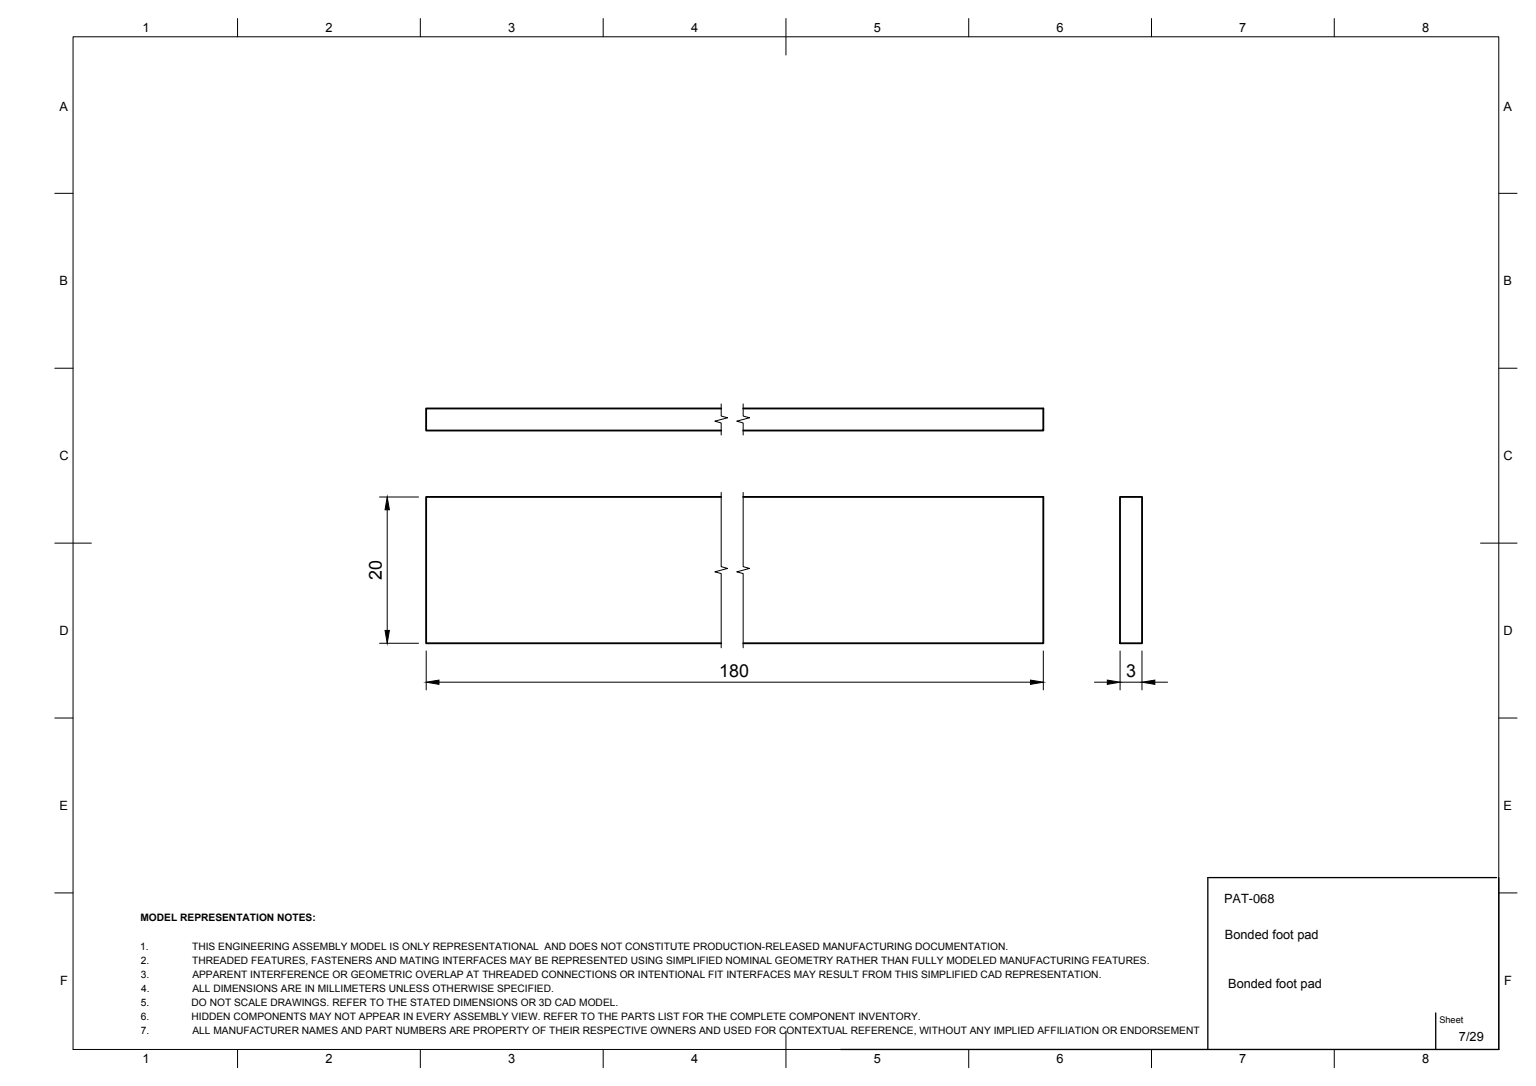
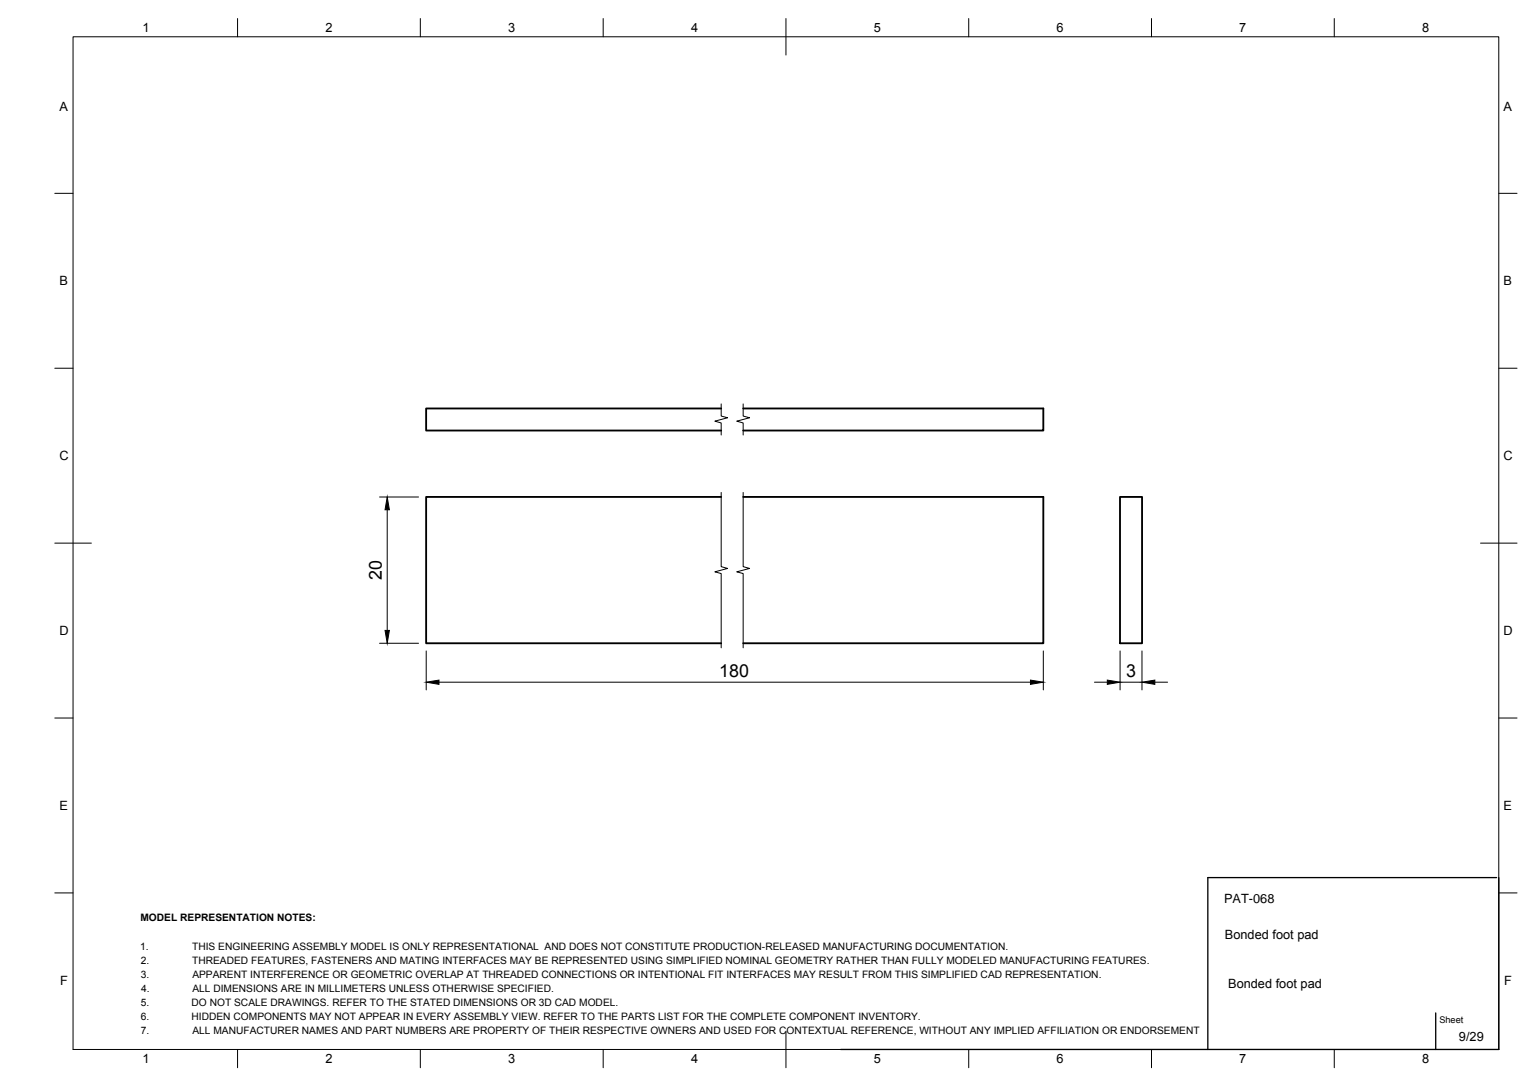
ISO-10303-21;
HEADER;
/* Generated by software containing ST-Developer
 * from STEP Tools, Inc. (www.steptools.com) 
 */

FILE_DESCRIPTION(
/* description */ ('Line shaft on three pillow blocks'),
/* implementation_level */ '2;1');

FILE_NAME(
/* name */ 'Bonded foot pad.step',
/* time_stamp */ '2026-10-27T10:49:19-07:00',
/* author */ (''),
/* organization */ (''),
/* preprocessor_version */ 'ST-DEVELOPER v20.2',
/* originating_system */ 'Autodesk Translation Framework v15.17.0.0',
/* authorisation */ '');

FILE_SCHEMA (('AUTOMOTIVE_DESIGN { 1 0 10303 214 3 1 1 }'));
ENDSEC;

DATA;
#10=MECHANICAL_DESIGN_GEOMETRIC_PRESENTATION_REPRESENTATION('',(#340),#8377);
#286=SHAPE_REPRESENTATION_RELATIONSHIP('SRR','None',#8501,#313);
#313=ADVANCED_BREP_SHAPE_REPRESENTATION('',(#368),#8350);
#340=STYLED_ITEM('',(#8711),#368);
#368=MANIFOLD_SOLID_BREP('Body1',#4326);
#502=PLANE('',#4708);
#503=PLANE('',#4709);
#504=PLANE('',#4710);
#505=PLANE('',#4711);
#506=PLANE('',#4712);
#507=PLANE('',#4713);
#680=FACE_OUTER_BOUND('',#954,.T.);
#681=FACE_OUTER_BOUND('',#955,.T.);
#682=FACE_OUTER_BOUND('',#956,.T.);
#683=FACE_OUTER_BOUND('',#957,.T.);
#684=FACE_OUTER_BOUND('',#958,.T.);
#685=FACE_OUTER_BOUND('',#959,.T.);
#954=EDGE_LOOP('',(#3069,#3070,#3071,#3072));
#955=EDGE_LOOP('',(#3073,#3074,#3075,#3076));
#956=EDGE_LOOP('',(#3077,#3078,#3079,#3080));
#957=EDGE_LOOP('',(#3081,#3082,#3083,#3084));
#958=EDGE_LOOP('',(#3085,#3086,#3087,#3088));
#959=EDGE_LOOP('',(#3089,#3090,#3091,#3092));
#1291=LINE('',#6599,#1618);
#1292=LINE('',#6601,#1619);
#1293=LINE('',#6603,#1620);
#1294=LINE('',#6604,#1621);
#1295=LINE('',#6607,#1622);
#1296=LINE('',#6609,#1623);
#1297=LINE('',#6610,#1624);
#1298=LINE('',#6613,#1625);
#1299=LINE('',#6615,#1626);
#1300=LINE('',#6616,#1627);
#1301=LINE('',#6618,#1628);
#1302=LINE('',#6619,#1629);
#1618=VECTOR('',#5296,1.);
#1619=VECTOR('',#5297,1.);
#1620=VECTOR('',#5298,1.);
#1621=VECTOR('',#5299,1.);
#1622=VECTOR('',#5302,1.);
#1623=VECTOR('',#5303,1.);
#1624=VECTOR('',#5304,1.);
#1625=VECTOR('',#5307,1.);
#1626=VECTOR('',#5308,1.);
#1627=VECTOR('',#5309,1.);
#1628=VECTOR('',#5312,1.);
#1629=VECTOR('',#5313,1.);
#2108=VERTEX_POINT('',#6597);
#2109=VERTEX_POINT('',#6598);
#2110=VERTEX_POINT('',#6600);
#2111=VERTEX_POINT('',#6602);
#2112=VERTEX_POINT('',#6606);
#2113=VERTEX_POINT('',#6608);
#2114=VERTEX_POINT('',#6612);
#2115=VERTEX_POINT('',#6614);
#2483=EDGE_CURVE('',#2108,#2109,#1291,.T.);
#2484=EDGE_CURVE('',#2109,#2110,#1292,.T.);
#2485=EDGE_CURVE('',#2111,#2110,#1293,.T.);
#2486=EDGE_CURVE('',#2108,#2111,#1294,.T.);
#2487=EDGE_CURVE('',#2112,#2108,#1295,.T.);
#2488=EDGE_CURVE('',#2113,#2111,#1296,.T.);
#2489=EDGE_CURVE('',#2112,#2113,#1297,.T.);
#2490=EDGE_CURVE('',#2114,#2112,#1298,.T.);
#2491=EDGE_CURVE('',#2115,#2113,#1299,.T.);
#2492=EDGE_CURVE('',#2114,#2115,#1300,.T.);
#2493=EDGE_CURVE('',#2109,#2114,#1301,.T.);
#2494=EDGE_CURVE('',#2110,#2115,#1302,.T.);
#3069=ORIENTED_EDGE('',*,*,#2483,.T.);
#3070=ORIENTED_EDGE('',*,*,#2484,.T.);
#3071=ORIENTED_EDGE('',*,*,#2485,.F.);
#3072=ORIENTED_EDGE('',*,*,#2486,.F.);
#3073=ORIENTED_EDGE('',*,*,#2487,.T.);
#3074=ORIENTED_EDGE('',*,*,#2486,.T.);
#3075=ORIENTED_EDGE('',*,*,#2488,.F.);
#3076=ORIENTED_EDGE('',*,*,#2489,.F.);
#3077=ORIENTED_EDGE('',*,*,#2490,.T.);
#3078=ORIENTED_EDGE('',*,*,#2489,.T.);
#3079=ORIENTED_EDGE('',*,*,#2491,.F.);
#3080=ORIENTED_EDGE('',*,*,#2492,.F.);
#3081=ORIENTED_EDGE('',*,*,#2493,.T.);
#3082=ORIENTED_EDGE('',*,*,#2492,.T.);
#3083=ORIENTED_EDGE('',*,*,#2494,.F.);
#3084=ORIENTED_EDGE('',*,*,#2484,.F.);
#3085=ORIENTED_EDGE('',*,*,#2494,.T.);
#3086=ORIENTED_EDGE('',*,*,#2491,.T.);
#3087=ORIENTED_EDGE('',*,*,#2488,.T.);
#3088=ORIENTED_EDGE('',*,*,#2485,.T.);
#3089=ORIENTED_EDGE('',*,*,#2493,.F.);
#3090=ORIENTED_EDGE('',*,*,#2483,.F.);
#3091=ORIENTED_EDGE('',*,*,#2487,.F.);
#3092=ORIENTED_EDGE('',*,*,#2490,.F.);
#4098=ADVANCED_FACE('',(#680),#502,.T.);
#4099=ADVANCED_FACE('',(#681),#503,.T.);
#4100=ADVANCED_FACE('',(#682),#504,.T.);
#4101=ADVANCED_FACE('',(#683),#505,.T.);
#4102=ADVANCED_FACE('',(#684),#506,.T.);
#4103=ADVANCED_FACE('',(#685),#507,.F.);
#4326=CLOSED_SHELL('',(#4098,#4099,#4100,#4101,#4102,#4103));
#4707=AXIS2_PLACEMENT_3D('',#6595,#5292,#5293);
#4708=AXIS2_PLACEMENT_3D('',#6596,#5294,#5295);
#4709=AXIS2_PLACEMENT_3D('',#6605,#5300,#5301);
#4710=AXIS2_PLACEMENT_3D('',#6611,#5305,#5306);
#4711=AXIS2_PLACEMENT_3D('',#6617,#5310,#5311);
#4712=AXIS2_PLACEMENT_3D('',#6620,#5314,#5315);
#4713=AXIS2_PLACEMENT_3D('',#6621,#5316,#5317);
#5292=DIRECTION('axis',(0.,0.,1.));
#5293=DIRECTION('refdir',(1.,0.,0.));
#5294=DIRECTION('center_axis',(0.,1.,0.));
#5295=DIRECTION('ref_axis',(-1.,0.,0.));
#5296=DIRECTION('',(-1.,0.,0.));
#5297=DIRECTION('',(0.,0.,1.));
#5298=DIRECTION('',(-1.,0.,0.));
#5299=DIRECTION('',(0.,0.,1.));
#5300=DIRECTION('center_axis',(1.,0.,0.));
#5301=DIRECTION('ref_axis',(0.,1.,0.));
#5302=DIRECTION('',(0.,1.,0.));
#5303=DIRECTION('',(0.,1.,0.));
#5304=DIRECTION('',(0.,0.,1.));
#5305=DIRECTION('center_axis',(0.,-1.,0.));
#5306=DIRECTION('ref_axis',(1.,0.,0.));
#5307=DIRECTION('',(1.,0.,0.));
#5308=DIRECTION('',(1.,0.,0.));
#5309=DIRECTION('',(0.,0.,1.));
#5310=DIRECTION('center_axis',(-1.,0.,0.));
#5311=DIRECTION('ref_axis',(0.,-1.,0.));
#5312=DIRECTION('',(0.,-1.,0.));
#5313=DIRECTION('',(0.,-1.,0.));
#5314=DIRECTION('center_axis',(0.,0.,1.));
#5315=DIRECTION('ref_axis',(1.,0.,0.));
#5316=DIRECTION('center_axis',(0.,0.,1.));
#5317=DIRECTION('ref_axis',(1.,0.,0.));
#6595=CARTESIAN_POINT('',(0.,0.,0.));
#6596=CARTESIAN_POINT('Origin',(9.,-2.,-1.8));
#6597=CARTESIAN_POINT('',(9.,-2.,-1.8));
#6598=CARTESIAN_POINT('',(-9.,-2.,-1.8));
#6599=CARTESIAN_POINT('',(9.,-2.,-1.8));
#6600=CARTESIAN_POINT('',(-9.,-2.,-1.5));
#6601=CARTESIAN_POINT('',(-9.,-2.,-1.8));
#6602=CARTESIAN_POINT('',(9.,-2.,-1.5));
#6603=CARTESIAN_POINT('',(9.,-2.,-1.5));
#6604=CARTESIAN_POINT('',(9.,-2.,-1.8));
#6605=CARTESIAN_POINT('Origin',(9.,-4.,-1.8));
#6606=CARTESIAN_POINT('',(9.,-4.,-1.8));
#6607=CARTESIAN_POINT('',(9.,-4.,-1.8));
#6608=CARTESIAN_POINT('',(9.,-4.,-1.5));
#6609=CARTESIAN_POINT('',(9.,-4.,-1.5));
#6610=CARTESIAN_POINT('',(9.,-4.,-1.8));
#6611=CARTESIAN_POINT('Origin',(-9.,-4.,-1.8));
#6612=CARTESIAN_POINT('',(-9.,-4.,-1.8));
#6613=CARTESIAN_POINT('',(-9.,-4.,-1.8));
#6614=CARTESIAN_POINT('',(-9.,-4.,-1.5));
#6615=CARTESIAN_POINT('',(-9.,-4.,-1.5));
#6616=CARTESIAN_POINT('',(-9.,-4.,-1.8));
#6617=CARTESIAN_POINT('Origin',(-9.,-2.,-1.8));
#6618=CARTESIAN_POINT('',(-9.,-2.,-1.8));
#6619=CARTESIAN_POINT('',(-9.,-2.,-1.5));
#6620=CARTESIAN_POINT('Origin',(0.,-3.,-1.5));
#6621=CARTESIAN_POINT('Origin',(0.,-3.,-1.8));
#8318=UNCERTAINTY_MEASURE_WITH_UNIT(LENGTH_MEASURE(0.001),#8378,
'DISTANCE_ACCURACY_VALUE',
'Maximum model space distance between geometric entities at asserted c
onnectivities');
#8345=UNCERTAINTY_MEASURE_WITH_UNIT(LENGTH_MEASURE(0.001),#8378,
'DISTANCE_ACCURACY_VALUE',
'Maximum model space distance between geometric entities at asserted c
onnectivities');
#8350=(
GEOMETRIC_REPRESENTATION_CONTEXT(3)
GLOBAL_UNCERTAINTY_ASSIGNED_CONTEXT((#8318))
GLOBAL_UNIT_ASSIGNED_CONTEXT((#8378,#8380,#8381))
REPRESENTATION_CONTEXT('','3D')
);
#8377=(
GEOMETRIC_REPRESENTATION_CONTEXT(3)
GLOBAL_UNCERTAINTY_ASSIGNED_CONTEXT((#8345))
GLOBAL_UNIT_ASSIGNED_CONTEXT((#8378,#8380,#8381))
REPRESENTATION_CONTEXT('','3D')
);
#8378=(
LENGTH_UNIT()
NAMED_UNIT(*)
SI_UNIT(.CENTI.,.METRE.)
);
#8380=(
NAMED_UNIT(*)
PLANE_ANGLE_UNIT()
SI_UNIT($,.RADIAN.)
);
#8381=(
NAMED_UNIT(*)
SI_UNIT($,.STERADIAN.)
SOLID_ANGLE_UNIT()
);
#8386=SHAPE_DEFINITION_REPRESENTATION(#8417,#8501);
#8417=PRODUCT_DEFINITION_SHAPE('',$,#8533);
#8501=SHAPE_REPRESENTATION('',(#4707),#8350);
#8528=PRODUCT_DEFINITION_CONTEXT('part definition',#8623,'design');
#8533=PRODUCT_DEFINITION('Bonded foot pad','Bonded foot pad',#8564,#8528);
#8564=PRODUCT_DEFINITION_FORMATION('',$,#8629);
#8623=APPLICATION_CONTEXT(
'Core Data for Automotive Mechanical Design Process');
#8624=PRODUCT_CONTEXT('part definition',#8623,'mechanical');
#8629=PRODUCT('Bonded foot pad','Bonded foot pad','Bonded foot pad',(#8624));
#8705=COLOUR_RGB('Sky Blue',0.24,0.69,0.87);
#8706=FILL_AREA_STYLE_COLOUR('',#8705);
#8707=FILL_AREA_STYLE('',(#8706));
#8708=SURFACE_STYLE_FILL_AREA(#8707);
#8709=SURFACE_SIDE_STYLE('',(#8708));
#8710=SURFACE_STYLE_USAGE(.BOTH.,#8709);
#8711=PRESENTATION_STYLE_ASSIGNMENT((#8710));
ENDSEC;
END-ISO-10303-21;
